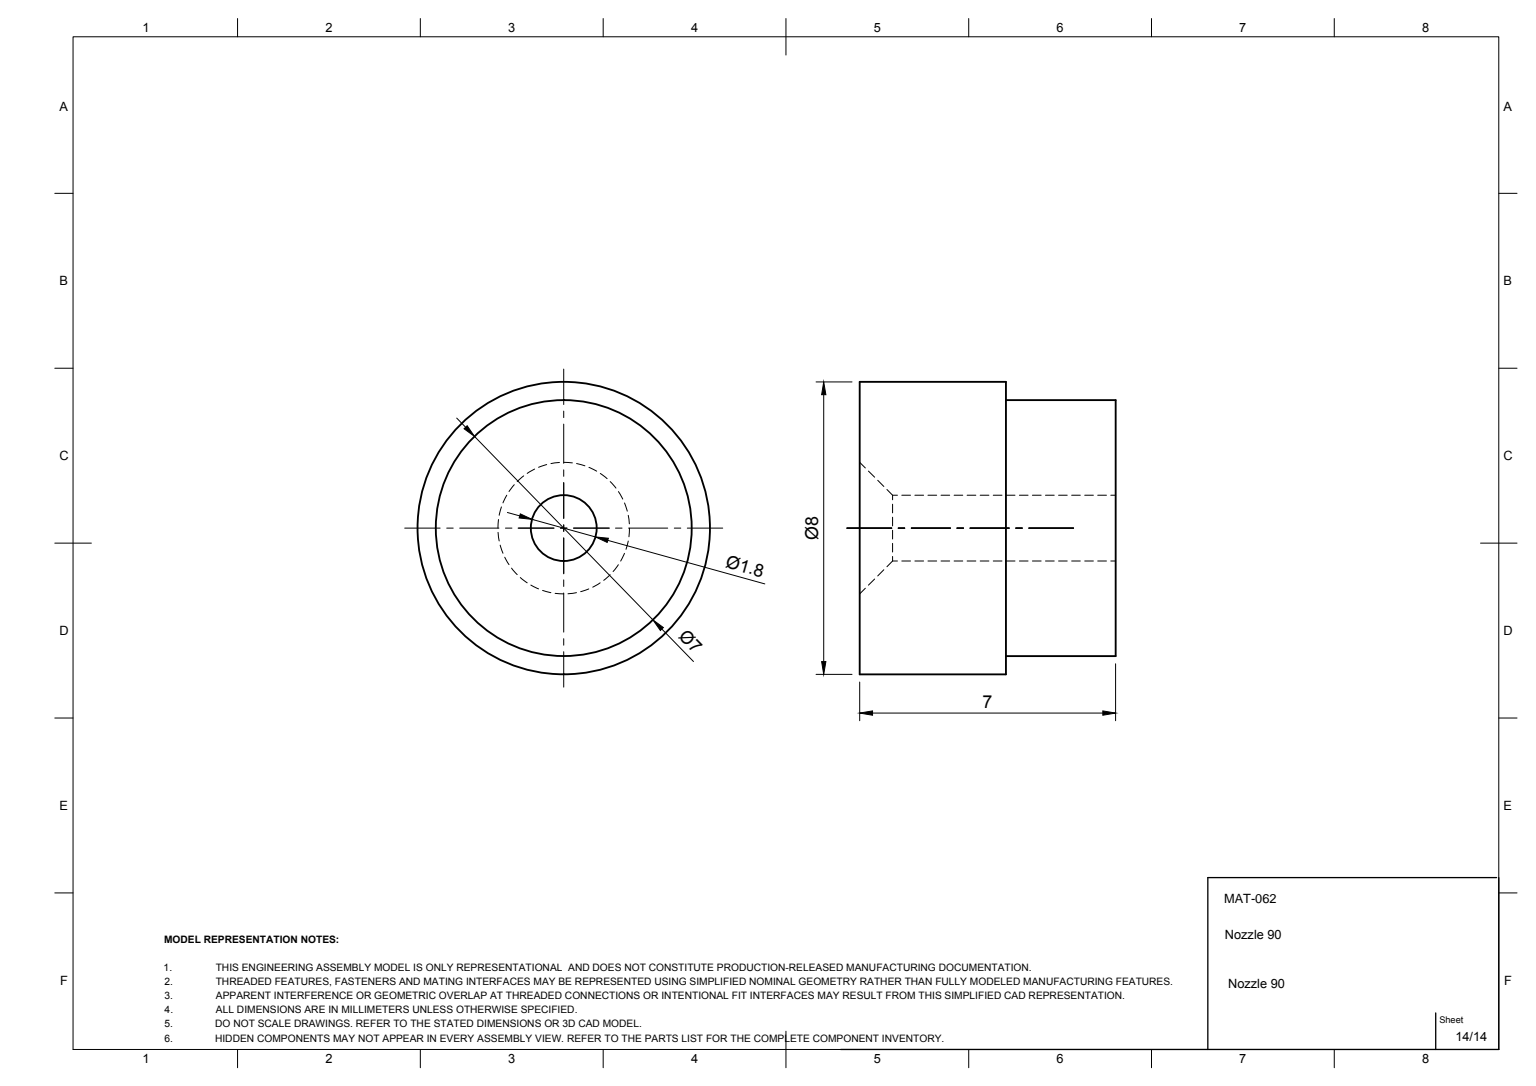
ISO-10303-21;
HEADER;
/* Generated by software containing ST-Developer
 * from STEP Tools, Inc. (www.steptools.com) 
 */

FILE_DESCRIPTION(
/* description */ (''),
/* implementation_level */ '2;1');

FILE_NAME(
/* name */ 'Nozzle 90.step',
/* time_stamp */ '2026-10-24T10:18:25-07:00',
/* author */ (''),
/* organization */ (''),
/* preprocessor_version */ 'ST-DEVELOPER v20.2',
/* originating_system */ 'Autodesk Translation Framework v15.15.0.0',
/* authorisation */ '');

FILE_SCHEMA (('AUTOMOTIVE_DESIGN { 1 0 10303 214 3 1 1 }'));
ENDSEC;

DATA;
#10=MECHANICAL_DESIGN_GEOMETRIC_PRESENTATION_REPRESENTATION('',(#263),#14125);
#197=CONICAL_SURFACE('',#6665,1.8,0.785398163397448);
#234=SHAPE_REPRESENTATION_RELATIONSHIP('SRR','None',#14208,#244);
#244=ADVANCED_BREP_SHAPE_REPRESENTATION('',(#276),#14122);
#263=STYLED_ITEM('',(#14263),#276);
#276=MANIFOLD_SOLID_BREP('Nozzle 90',#6144);
#563=CYLINDRICAL_SURFACE('',#6655,4.00000000000013);
#564=CYLINDRICAL_SURFACE('',#6662,0.899999999999984);
#565=CYLINDRICAL_SURFACE('',#6668,3.50000000000012);
#684=FACE_BOUND('',#1372,.T.);
#685=FACE_BOUND('',#1374,.T.);
#686=FACE_BOUND('',#1378,.T.);
#960=FACE_OUTER_BOUND('',#1370,.T.);
#961=FACE_OUTER_BOUND('',#1371,.T.);
#962=FACE_OUTER_BOUND('',#1373,.T.);
#963=FACE_OUTER_BOUND('',#1375,.T.);
#964=FACE_OUTER_BOUND('',#1376,.T.);
#965=FACE_OUTER_BOUND('',#1377,.T.);
#966=FACE_OUTER_BOUND('',#1379,.T.);
#1370=EDGE_LOOP('',(#5047,#5048,#5049,#5050));
#1371=EDGE_LOOP('',(#5051));
#1372=EDGE_LOOP('',(#5052));
#1373=EDGE_LOOP('',(#5053));
#1374=EDGE_LOOP('',(#5054));
#1375=EDGE_LOOP('',(#5055,#5056,#5057,#5058));
#1376=EDGE_LOOP('',(#5059,#5060,#5061,#5062));
#1377=EDGE_LOOP('',(#5063));
#1378=EDGE_LOOP('',(#5064));
#1379=EDGE_LOOP('',(#5065,#5066,#5067,#5068));
#1720=CIRCLE('',#6656,4.00000000000013);
#1721=CIRCLE('',#6657,4.00000000000013);
#1722=CIRCLE('',#6659,3.50000000000012);
#1723=CIRCLE('',#6661,1.8);
#1724=CIRCLE('',#6663,0.89999999999999);
#1725=CIRCLE('',#6664,0.899999999999984);
#1726=CIRCLE('',#6667,3.50000000000012);
#2050=LINE('',#12296,#2438);
#2051=LINE('',#12308,#2439);
#2052=LINE('',#12311,#2440);
#2053=LINE('',#12316,#2441);
#2438=VECTOR('',#7952,4.00000000000013);
#2439=VECTOR('',#7967,0.899999999999984);
#2440=VECTOR('',#7972,1.8);
#2441=VECTOR('',#7979,3.50000000000012);
#2937=VERTEX_POINT('',#12293);
#2938=VERTEX_POINT('',#12295);
#2939=VERTEX_POINT('',#12299);
#2940=VERTEX_POINT('',#12302);
#2941=VERTEX_POINT('',#12305);
#2942=VERTEX_POINT('',#12307);
#2943=VERTEX_POINT('',#12313);
#3671=EDGE_CURVE('',#2937,#2937,#1720,.T.);
#3672=EDGE_CURVE('',#2937,#2938,#2050,.T.);
#3673=EDGE_CURVE('',#2938,#2938,#1721,.T.);
#3674=EDGE_CURVE('',#2939,#2939,#1722,.T.);
#3675=EDGE_CURVE('',#2940,#2940,#1723,.T.);
#3676=EDGE_CURVE('',#2941,#2941,#1724,.T.);
#3677=EDGE_CURVE('',#2941,#2942,#2051,.T.);
#3678=EDGE_CURVE('',#2942,#2942,#1725,.T.);
#3679=EDGE_CURVE('',#2942,#2940,#2052,.T.);
#3680=EDGE_CURVE('',#2943,#2943,#1726,.T.);
#3681=EDGE_CURVE('',#2939,#2943,#2053,.T.);
#5047=ORIENTED_EDGE('',*,*,#3671,.F.);
#5048=ORIENTED_EDGE('',*,*,#3672,.T.);
#5049=ORIENTED_EDGE('',*,*,#3673,.T.);
#5050=ORIENTED_EDGE('',*,*,#3672,.F.);
#5051=ORIENTED_EDGE('',*,*,#3673,.F.);
#5052=ORIENTED_EDGE('',*,*,#3674,.F.);
#5053=ORIENTED_EDGE('',*,*,#3671,.T.);
#5054=ORIENTED_EDGE('',*,*,#3675,.F.);
#5055=ORIENTED_EDGE('',*,*,#3676,.F.);
#5056=ORIENTED_EDGE('',*,*,#3677,.T.);
#5057=ORIENTED_EDGE('',*,*,#3678,.T.);
#5058=ORIENTED_EDGE('',*,*,#3677,.F.);
#5059=ORIENTED_EDGE('',*,*,#3678,.F.);
#5060=ORIENTED_EDGE('',*,*,#3679,.T.);
#5061=ORIENTED_EDGE('',*,*,#3675,.T.);
#5062=ORIENTED_EDGE('',*,*,#3679,.F.);
#5063=ORIENTED_EDGE('',*,*,#3680,.T.);
#5064=ORIENTED_EDGE('',*,*,#3676,.T.);
#5065=ORIENTED_EDGE('',*,*,#3674,.T.);
#5066=ORIENTED_EDGE('',*,*,#3681,.T.);
#5067=ORIENTED_EDGE('',*,*,#3680,.F.);
#5068=ORIENTED_EDGE('',*,*,#3681,.F.);
#5725=PLANE('',#6658);
#5726=PLANE('',#6660);
#5727=PLANE('',#6666);
#6009=ADVANCED_FACE('',(#960),#563,.T.);
#6010=ADVANCED_FACE('',(#961,#684),#5725,.F.);
#6011=ADVANCED_FACE('',(#962,#685),#5726,.T.);
#6012=ADVANCED_FACE('',(#963),#564,.F.);
#6013=ADVANCED_FACE('',(#964),#197,.F.);
#6014=ADVANCED_FACE('',(#965,#686),#5727,.T.);
#6015=ADVANCED_FACE('',(#966),#565,.T.);
#6144=CLOSED_SHELL('',(#6009,#6010,#6011,#6012,#6013,#6014,#6015));
#6654=AXIS2_PLACEMENT_3D('',#12291,#7946,#7947);
#6655=AXIS2_PLACEMENT_3D('',#12292,#7948,#7949);
#6656=AXIS2_PLACEMENT_3D('',#12294,#7950,#7951);
#6657=AXIS2_PLACEMENT_3D('',#12297,#7953,#7954);
#6658=AXIS2_PLACEMENT_3D('',#12298,#7955,#7956);
#6659=AXIS2_PLACEMENT_3D('',#12300,#7957,#7958);
#6660=AXIS2_PLACEMENT_3D('',#12301,#7959,#7960);
#6661=AXIS2_PLACEMENT_3D('',#12303,#7961,#7962);
#6662=AXIS2_PLACEMENT_3D('',#12304,#7963,#7964);
#6663=AXIS2_PLACEMENT_3D('',#12306,#7965,#7966);
#6664=AXIS2_PLACEMENT_3D('',#12309,#7968,#7969);
#6665=AXIS2_PLACEMENT_3D('',#12310,#7970,#7971);
#6666=AXIS2_PLACEMENT_3D('',#12312,#7973,#7974);
#6667=AXIS2_PLACEMENT_3D('',#12314,#7975,#7976);
#6668=AXIS2_PLACEMENT_3D('',#12315,#7977,#7978);
#7946=DIRECTION('axis',(0.,0.,1.));
#7947=DIRECTION('refdir',(1.,0.,0.));
#7948=DIRECTION('center_axis',(0.,1.,0.));
#7949=DIRECTION('ref_axis',(0.,0.,1.));
#7950=DIRECTION('center_axis',(0.,1.,0.));
#7951=DIRECTION('ref_axis',(0.,0.,1.));
#7952=DIRECTION('',(0.,-1.,0.));
#7953=DIRECTION('center_axis',(0.,1.,0.));
#7954=DIRECTION('ref_axis',(0.,0.,1.));
#7955=DIRECTION('center_axis',(0.,1.,0.));
#7956=DIRECTION('ref_axis',(0.,0.,1.));
#7957=DIRECTION('center_axis',(0.,-1.,0.));
#7958=DIRECTION('ref_axis',(0.,0.,-1.));
#7959=DIRECTION('center_axis',(0.,1.,0.));
#7960=DIRECTION('ref_axis',(0.,0.,1.));
#7961=DIRECTION('center_axis',(0.,1.,0.));
#7962=DIRECTION('ref_axis',(0.,0.,1.));
#7963=DIRECTION('center_axis',(0.,1.,0.));
#7964=DIRECTION('ref_axis',(0.,0.,1.));
#7965=DIRECTION('center_axis',(0.,1.,0.));
#7966=DIRECTION('ref_axis',(0.,0.,1.));
#7967=DIRECTION('',(0.,1.,0.));
#7968=DIRECTION('center_axis',(0.,1.,0.));
#7969=DIRECTION('ref_axis',(0.,0.,1.));
#7970=DIRECTION('center_axis',(0.,1.,0.));
#7971=DIRECTION('ref_axis',(0.,0.,1.));
#7972=DIRECTION('',(-8.65956056235494E-17,0.707106781186548,-0.707106781186548));
#7973=DIRECTION('center_axis',(0.,-1.,0.));
#7974=DIRECTION('ref_axis',(0.,0.,-1.));
#7975=DIRECTION('center_axis',(0.,-1.,0.));
#7976=DIRECTION('ref_axis',(0.,0.,-1.));
#7977=DIRECTION('center_axis',(0.,1.,0.));
#7978=DIRECTION('ref_axis',(0.,0.,1.));
#7979=DIRECTION('',(0.,-1.,0.));
#12291=CARTESIAN_POINT('',(0.,0.,0.));
#12292=CARTESIAN_POINT('Origin',(-75.5607164801933,132.,-55.624999999998));
#12293=CARTESIAN_POINT('',(-75.5607164801933,136.,-59.6249999999981));
#12294=CARTESIAN_POINT('Origin',(-75.5607164801933,136.,-55.624999999998));
#12295=CARTESIAN_POINT('',(-75.5607164801933,132.,-59.6249999999981));
#12296=CARTESIAN_POINT('',(-75.5607164801933,132.,-59.6249999999981));
#12297=CARTESIAN_POINT('Origin',(-75.5607164801933,132.,-55.624999999998));
#12298=CARTESIAN_POINT('Origin',(-75.5607164801933,132.,-55.624999999998));
#12299=CARTESIAN_POINT('',(-75.5607164801933,132.,-59.1249999999981));
#12300=CARTESIAN_POINT('Origin',(-75.5607164801933,132.,-55.624999999998));
#12301=CARTESIAN_POINT('Origin',(-75.5607164801933,136.,-55.624999999998));
#12302=CARTESIAN_POINT('',(-75.5607164801933,136.,-57.424999999998));
#12303=CARTESIAN_POINT('Origin',(-75.5607164801933,136.,-55.624999999998));
#12304=CARTESIAN_POINT('Origin',(-75.5607164801933,136.,-55.624999999998));
#12305=CARTESIAN_POINT('',(-75.5607164801933,129.,-56.524999999998));
#12306=CARTESIAN_POINT('Origin',(-75.5607164801933,129.,-55.624999999998));
#12307=CARTESIAN_POINT('',(-75.5607164801933,135.1,-56.524999999998));
#12308=CARTESIAN_POINT('',(-75.5607164801933,136.,-56.524999999998));
#12309=CARTESIAN_POINT('Origin',(-75.5607164801933,135.1,-55.624999999998));
#12310=CARTESIAN_POINT('Origin',(-75.5607164801933,136.,-55.624999999998));
#12311=CARTESIAN_POINT('',(-75.5607164801933,136.,-57.424999999998));
#12312=CARTESIAN_POINT('Origin',(-75.5607164801933,129.,-55.624999999998));
#12313=CARTESIAN_POINT('',(-75.5607164801933,129.,-59.1249999999981));
#12314=CARTESIAN_POINT('Origin',(-75.5607164801933,129.,-55.624999999998));
#12315=CARTESIAN_POINT('Origin',(-75.5607164801933,129.,-55.624999999998));
#12316=CARTESIAN_POINT('',(-75.5607164801933,129.,-59.1249999999981));
#14109=UNCERTAINTY_MEASURE_WITH_UNIT(LENGTH_MEASURE(0.01),#14126,
'DISTANCE_ACCURACY_VALUE',
'Maximum model space distance between geometric entities at asserted c
onnectivities');
#14112=UNCERTAINTY_MEASURE_WITH_UNIT(LENGTH_MEASURE(0.01),#14126,
'DISTANCE_ACCURACY_VALUE',
'Maximum model space distance between geometric entities at asserted c
onnectivities');
#14122=(
GEOMETRIC_REPRESENTATION_CONTEXT(3)
GLOBAL_UNCERTAINTY_ASSIGNED_CONTEXT((#14109))
GLOBAL_UNIT_ASSIGNED_CONTEXT((#14126,#14128,#14129))
REPRESENTATION_CONTEXT('','3D')
);
#14125=(
GEOMETRIC_REPRESENTATION_CONTEXT(3)
GLOBAL_UNCERTAINTY_ASSIGNED_CONTEXT((#14112))
GLOBAL_UNIT_ASSIGNED_CONTEXT((#14126,#14128,#14129))
REPRESENTATION_CONTEXT('','3D')
);
#14126=(
LENGTH_UNIT()
NAMED_UNIT(*)
SI_UNIT(.MILLI.,.METRE.)
);
#14128=(
NAMED_UNIT(*)
PLANE_ANGLE_UNIT()
SI_UNIT($,.RADIAN.)
);
#14129=(
NAMED_UNIT(*)
SI_UNIT($,.STERADIAN.)
SOLID_ANGLE_UNIT()
);
#14139=SHAPE_DEFINITION_REPRESENTATION(#14151,#14208);
#14151=PRODUCT_DEFINITION_SHAPE('',$,#14221);
#14208=SHAPE_REPRESENTATION('',(#6654),#14122);
#14211=PRODUCT_DEFINITION_CONTEXT('part definition',#14249,'design');
#14221=PRODUCT_DEFINITION('Nozzle 90','Nozzle 90',#14233,#14211);
#14233=PRODUCT_DEFINITION_FORMATION('',$,#14260);
#14249=APPLICATION_CONTEXT(
'Core Data for Automotive Mechanical Design Process');
#14250=PRODUCT_CONTEXT('part definition',#14249,'mechanical');
#14260=PRODUCT('Nozzle 90','Nozzle 90',$,(#14250));
#14263=PRESENTATION_STYLE_ASSIGNMENT((#14265));
#14265=SURFACE_STYLE_USAGE(.BOTH.,#14267);
#14267=SURFACE_SIDE_STYLE('',(#14269));
#14269=SURFACE_STYLE_FILL_AREA(#14271);
#14271=FILL_AREA_STYLE('Steel - Satin',(#14273));
#14273=FILL_AREA_STYLE_COLOUR('Steel - Satin',#14275);
#14275=COLOUR_RGB('Steel - Satin',0.627450980392157,0.627450980392157,0.627450980392157);
ENDSEC;
END-ISO-10303-21;
